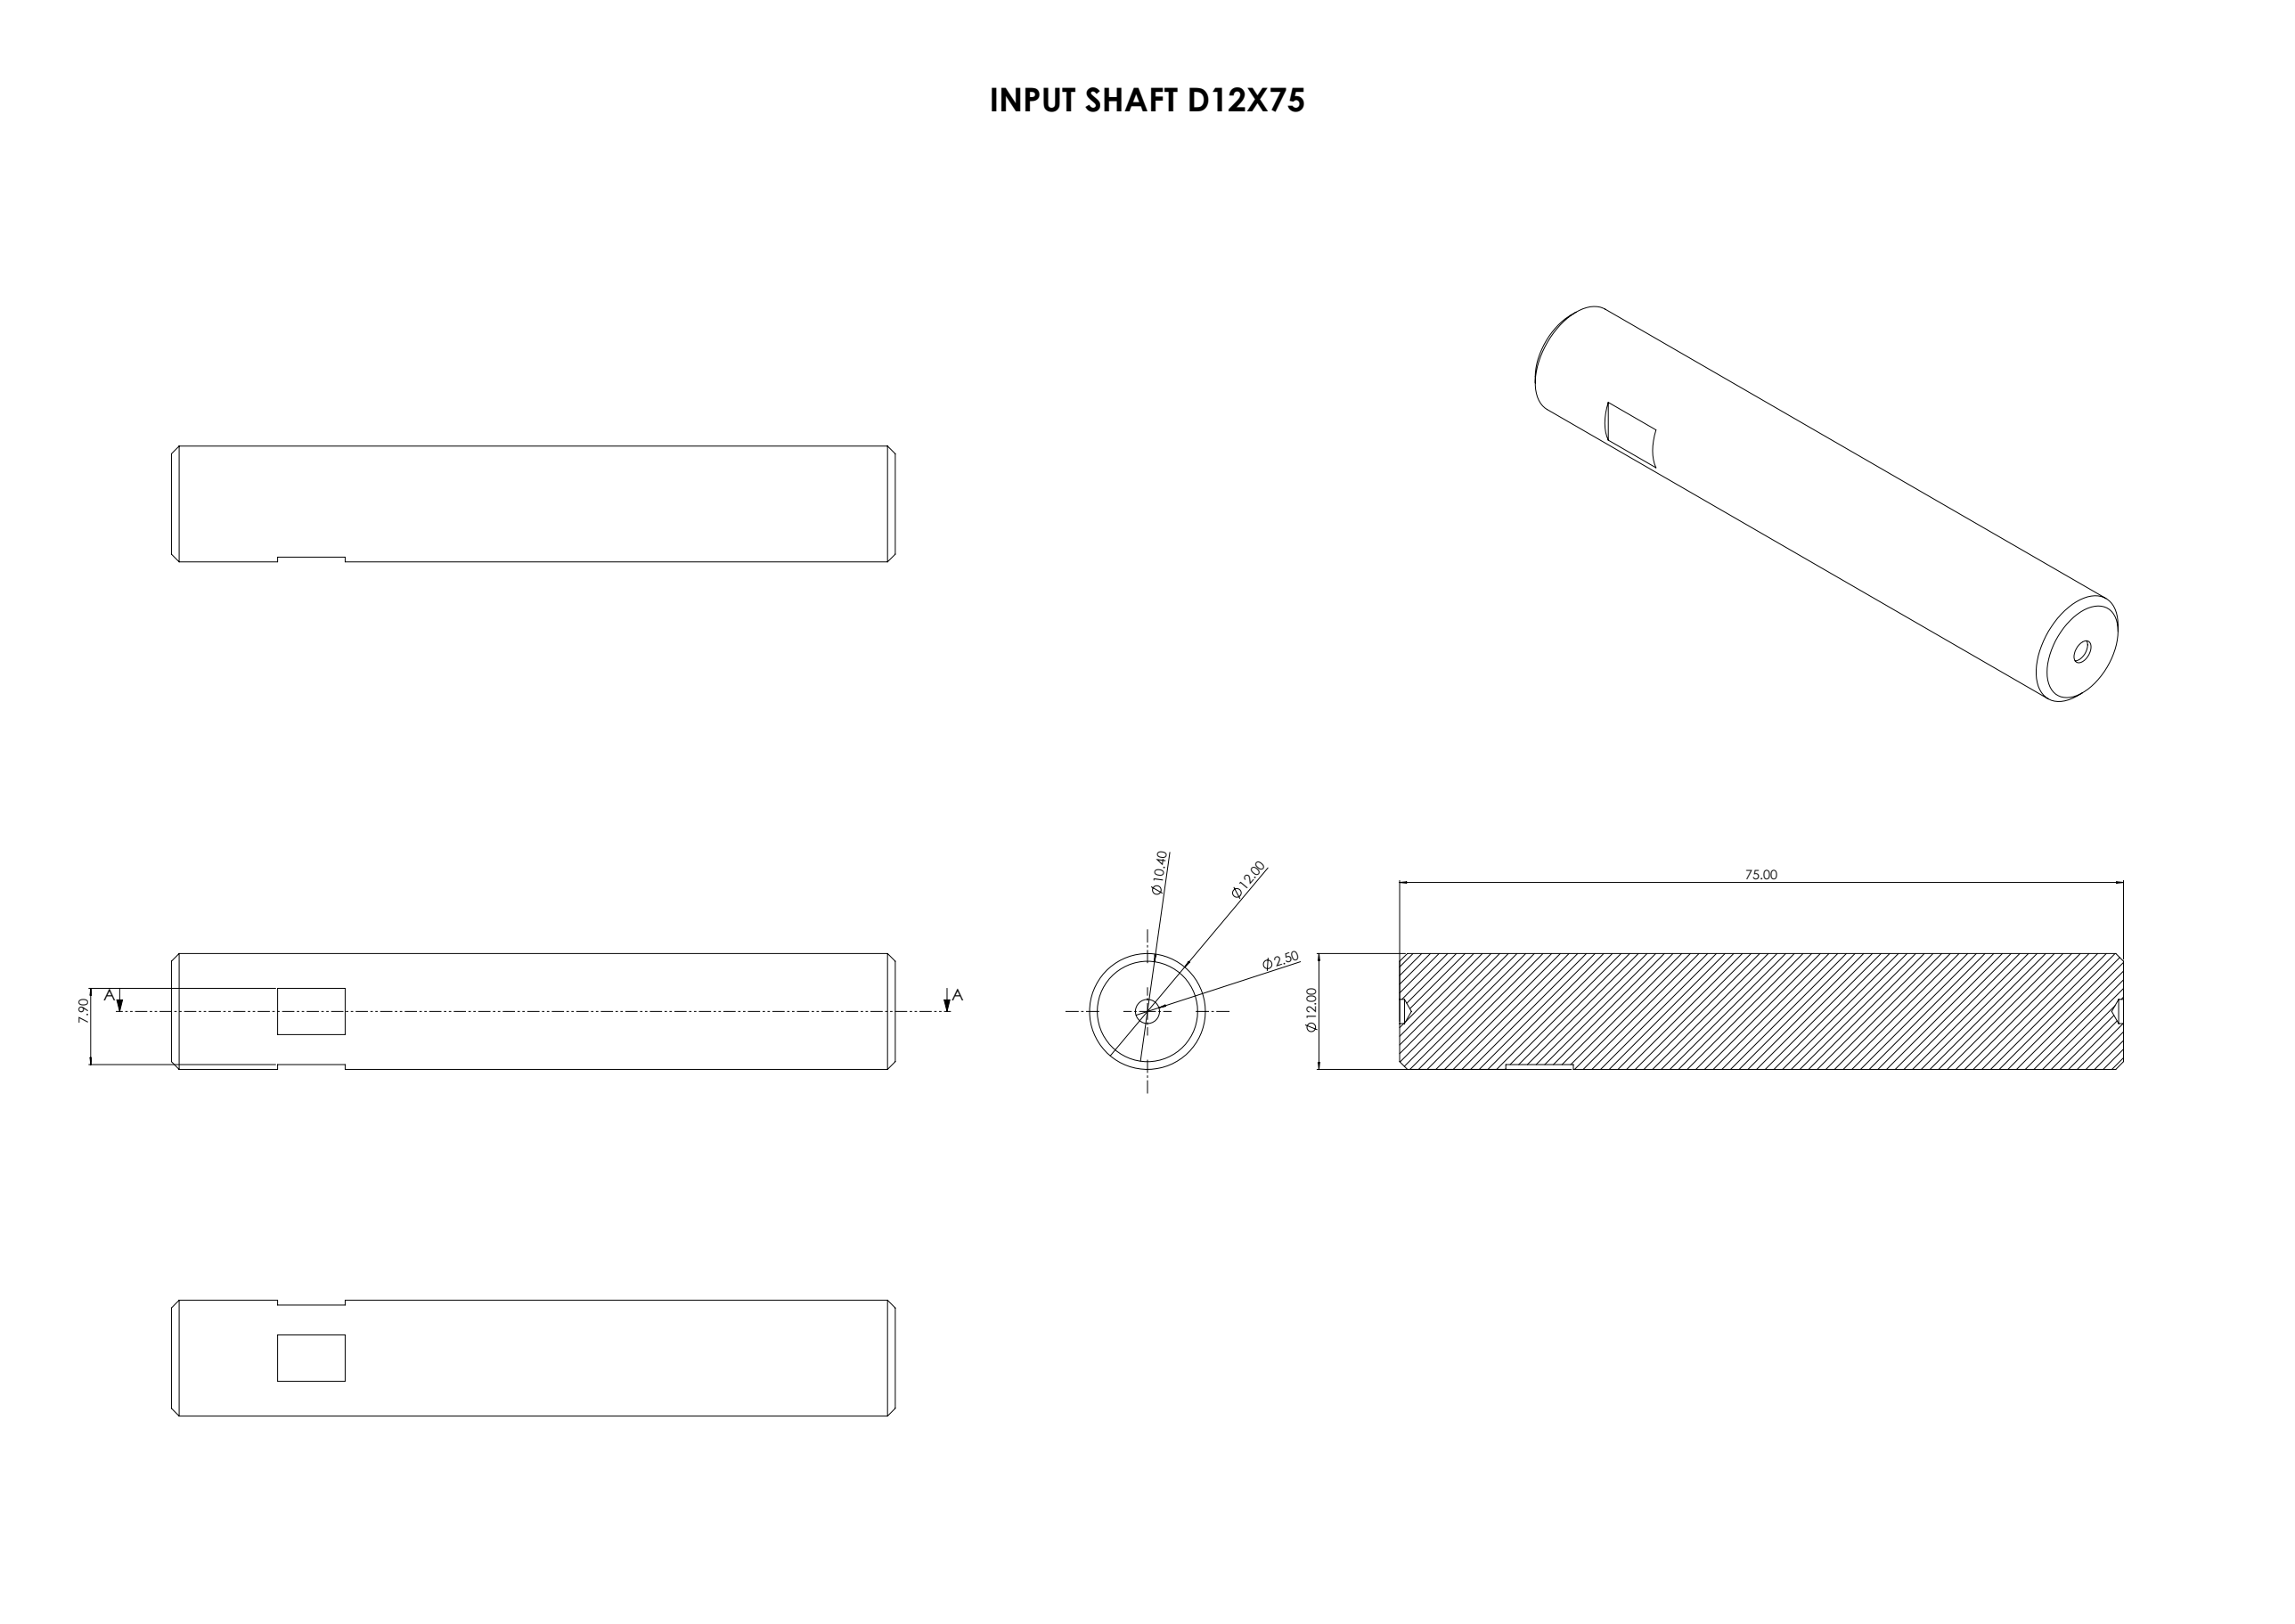
ISO-10303-21;
HEADER;
/* Generated by software containing ST-Developer
 * from STEP Tools, Inc. (www.steptools.com) 
 */

FILE_DESCRIPTION(
/* description */ (''),
/* implementation_level */ '2;1');

FILE_NAME(
/* name */ '04_Input_Shaft_D12x75.step',
/* time_stamp */ '2026-10-11T09:12:28-07:00',
/* author */ (''),
/* organization */ (''),
/* preprocessor_version */ 'ST-DEVELOPER v20.2',
/* originating_system */ 'Autodesk Translation Framework v15.15.0.0',
/* authorisation */ '');

FILE_SCHEMA (('AUTOMOTIVE_DESIGN { 1 0 10303 214 3 1 1 }'));
ENDSEC;

DATA;
#10=MECHANICAL_DESIGN_GEOMETRIC_PRESENTATION_REPRESENTATION('',(#650),#23254);
#630=SHAPE_REPRESENTATION_RELATIONSHIP('SRR','None',#23303,#640);
#640=ADVANCED_BREP_SHAPE_REPRESENTATION('',(#660),#23247);
#650=STYLED_ITEM('',(#23462),#660);
#660=MANIFOLD_SOLID_BREP('Body1',#7028);
#735=CONICAL_SURFACE('',#7557,0.625,1.04746029293308);
#736=CONICAL_SURFACE('',#7564,1.25,1.04746029293308);
#737=CONICAL_SURFACE('',#7567,5.6,0.785398163397448);
#738=CONICAL_SURFACE('',#7571,5.6,0.785398163397448);
#808=FACE_BOUND('',#1674,.T.);
#809=FACE_BOUND('',#1677,.T.);
#810=FACE_BOUND('',#1680,.T.);
#932=PLANE('',#7545);
#933=PLANE('',#7548);
#934=PLANE('',#7551);
#935=PLANE('',#7552);
#936=PLANE('',#7554);
#937=PLANE('',#7555);
#938=PLANE('',#7565);
#939=PLANE('',#7573);
#1240=FACE_OUTER_BOUND('',#1663,.T.);
#1241=FACE_OUTER_BOUND('',#1664,.T.);
#1242=FACE_OUTER_BOUND('',#1665,.T.);
#1243=FACE_OUTER_BOUND('',#1666,.T.);
#1244=FACE_OUTER_BOUND('',#1667,.T.);
#1245=FACE_OUTER_BOUND('',#1668,.T.);
#1246=FACE_OUTER_BOUND('',#1669,.T.);
#1247=FACE_OUTER_BOUND('',#1670,.T.);
#1248=FACE_OUTER_BOUND('',#1671,.T.);
#1249=FACE_OUTER_BOUND('',#1672,.T.);
#1250=FACE_OUTER_BOUND('',#1673,.T.);
#1251=FACE_OUTER_BOUND('',#1675,.T.);
#1252=FACE_OUTER_BOUND('',#1676,.T.);
#1253=FACE_OUTER_BOUND('',#1678,.T.);
#1254=FACE_OUTER_BOUND('',#1679,.T.);
#1663=EDGE_LOOP('',(#5873,#5874,#5875));
#1664=EDGE_LOOP('',(#5876,#5877,#5878));
#1665=EDGE_LOOP('',(#5879,#5880,#5881,#5882));
#1666=EDGE_LOOP('',(#5883,#5884));
#1667=EDGE_LOOP('',(#5885,#5886,#5887,#5888));
#1668=EDGE_LOOP('',(#5889,#5890));
#1669=EDGE_LOOP('',(#5891,#5892,#5893));
#1670=EDGE_LOOP('',(#5894,#5895,#5896,#5897));
#1671=EDGE_LOOP('',(#5898,#5899,#5900,#5901));
#1672=EDGE_LOOP('',(#5902,#5903,#5904));
#1673=EDGE_LOOP('',(#5905));
#1674=EDGE_LOOP('',(#5906));
#1675=EDGE_LOOP('',(#5907,#5908,#5909,#5910));
#1676=EDGE_LOOP('',(#5911,#5912,#5913,#5914,#5915,#5916,#5917,#5918,#5919,
#5920,#5921,#5922));
#1677=EDGE_LOOP('',(#5923,#5924,#5925,#5926));
#1678=EDGE_LOOP('',(#5927,#5928,#5929,#5930));
#1679=EDGE_LOOP('',(#5931));
#1680=EDGE_LOOP('',(#5932));
#1993=LINE('',#20982,#2252);
#1994=LINE('',#20989,#2253);
#1995=LINE('',#20992,#2254);
#1996=LINE('',#20993,#2255);
#1997=LINE('',#20998,#2256);
#1998=LINE('',#21001,#2257);
#1999=LINE('',#21003,#2258);
#2000=LINE('',#21004,#2259);
#2001=LINE('',#21010,#2260);
#2002=LINE('',#21014,#2261);
#2003=LINE('',#21020,#2262);
#2004=LINE('',#21024,#2263);
#2005=LINE('',#21031,#2264);
#2006=LINE('',#21035,#2265);
#2007=LINE('',#21036,#2266);
#2008=LINE('',#21040,#2267);
#2252=VECTOR('',#8785,10.);
#2253=VECTOR('',#8792,10.);
#2254=VECTOR('',#8797,10.);
#2255=VECTOR('',#8798,10.);
#2256=VECTOR('',#8803,10.);
#2257=VECTOR('',#8806,10.);
#2258=VECTOR('',#8807,10.);
#2259=VECTOR('',#8808,10.);
#2260=VECTOR('',#8815,0.625);
#2261=VECTOR('',#8820,1.25);
#2262=VECTOR('',#8827,1.25);
#2263=VECTOR('',#8832,1.25);
#2264=VECTOR('',#8841,5.6);
#2265=VECTOR('',#8846,6.);
#2266=VECTOR('',#8847,6.);
#2267=VECTOR('',#8852,5.6);
#2572=CIRCLE('',#7546,6.);
#2573=CIRCLE('',#7547,6.);
#2574=CIRCLE('',#7549,6.);
#2575=CIRCLE('',#7550,6.);
#2576=CIRCLE('',#7553,6.);
#2577=CIRCLE('',#7556,6.);
#2578=CIRCLE('',#7558,1.25);
#2579=CIRCLE('',#7560,1.25);
#2580=CIRCLE('',#7562,1.25);
#2581=CIRCLE('',#7563,1.25);
#2582=CIRCLE('',#7566,5.2);
#2583=CIRCLE('',#7568,6.);
#2584=CIRCLE('',#7570,6.);
#2585=CIRCLE('',#7572,5.2);
#3164=VERTEX_POINT('',#20978);
#3165=VERTEX_POINT('',#20979);
#3166=VERTEX_POINT('',#20981);
#3167=VERTEX_POINT('',#20985);
#3168=VERTEX_POINT('',#20986);
#3169=VERTEX_POINT('',#20988);
#3170=VERTEX_POINT('',#20995);
#3171=VERTEX_POINT('',#20996);
#3172=VERTEX_POINT('',#21000);
#3173=VERTEX_POINT('',#21002);
#3174=VERTEX_POINT('',#21008);
#3175=VERTEX_POINT('',#21009);
#3176=VERTEX_POINT('',#21013);
#3177=VERTEX_POINT('',#21017);
#3178=VERTEX_POINT('',#21019);
#3179=VERTEX_POINT('',#21023);
#3180=VERTEX_POINT('',#21026);
#3181=VERTEX_POINT('',#21029);
#3182=VERTEX_POINT('',#21033);
#3183=VERTEX_POINT('',#21038);
#4112=EDGE_CURVE('',#3164,#3165,#2572,.T.);
#4113=EDGE_CURVE('',#3164,#3166,#1993,.T.);
#4114=EDGE_CURVE('',#3165,#3166,#2573,.T.);
#4115=EDGE_CURVE('',#3167,#3168,#2574,.T.);
#4116=EDGE_CURVE('',#3167,#3169,#1994,.T.);
#4117=EDGE_CURVE('',#3168,#3169,#2575,.T.);
#4118=EDGE_CURVE('',#3169,#3164,#1995,.T.);
#4119=EDGE_CURVE('',#3166,#3167,#1996,.T.);
#4120=EDGE_CURVE('',#3170,#3171,#2576,.T.);
#4121=EDGE_CURVE('',#3170,#3171,#1997,.T.);
#4122=EDGE_CURVE('',#3172,#3170,#1998,.T.);
#4123=EDGE_CURVE('',#3173,#3172,#1999,.T.);
#4124=EDGE_CURVE('',#3171,#3173,#2000,.T.);
#4125=EDGE_CURVE('',#3173,#3172,#2577,.T.);
#4126=EDGE_CURVE('',#3174,#3175,#2001,.T.);
#4127=EDGE_CURVE('',#3175,#3175,#2578,.T.);
#4128=EDGE_CURVE('',#3175,#3176,#2002,.T.);
#4129=EDGE_CURVE('',#3176,#3176,#2579,.T.);
#4130=EDGE_CURVE('',#3177,#3177,#2580,.T.);
#4131=EDGE_CURVE('',#3177,#3178,#2003,.T.);
#4132=EDGE_CURVE('',#3178,#3178,#2581,.T.);
#4133=EDGE_CURVE('',#3178,#3179,#2004,.T.);
#4134=EDGE_CURVE('',#3180,#3180,#2582,.T.);
#4135=EDGE_CURVE('',#3181,#3181,#2583,.T.);
#4136=EDGE_CURVE('',#3181,#3180,#2005,.T.);
#4137=EDGE_CURVE('',#3182,#3182,#2584,.T.);
#4138=EDGE_CURVE('',#3182,#3168,#2006,.T.);
#4139=EDGE_CURVE('',#3165,#3181,#2007,.T.);
#4140=EDGE_CURVE('',#3183,#3183,#2585,.T.);
#4141=EDGE_CURVE('',#3183,#3182,#2008,.T.);
#5873=ORIENTED_EDGE('',*,*,#4112,.F.);
#5874=ORIENTED_EDGE('',*,*,#4113,.T.);
#5875=ORIENTED_EDGE('',*,*,#4114,.F.);
#5876=ORIENTED_EDGE('',*,*,#4115,.F.);
#5877=ORIENTED_EDGE('',*,*,#4116,.T.);
#5878=ORIENTED_EDGE('',*,*,#4117,.F.);
#5879=ORIENTED_EDGE('',*,*,#4118,.F.);
#5880=ORIENTED_EDGE('',*,*,#4116,.F.);
#5881=ORIENTED_EDGE('',*,*,#4119,.F.);
#5882=ORIENTED_EDGE('',*,*,#4113,.F.);
#5883=ORIENTED_EDGE('',*,*,#4120,.F.);
#5884=ORIENTED_EDGE('',*,*,#4121,.T.);
#5885=ORIENTED_EDGE('',*,*,#4122,.F.);
#5886=ORIENTED_EDGE('',*,*,#4123,.F.);
#5887=ORIENTED_EDGE('',*,*,#4124,.F.);
#5888=ORIENTED_EDGE('',*,*,#4121,.F.);
#5889=ORIENTED_EDGE('',*,*,#4125,.F.);
#5890=ORIENTED_EDGE('',*,*,#4123,.T.);
#5891=ORIENTED_EDGE('',*,*,#4126,.T.);
#5892=ORIENTED_EDGE('',*,*,#4127,.T.);
#5893=ORIENTED_EDGE('',*,*,#4126,.F.);
#5894=ORIENTED_EDGE('',*,*,#4127,.F.);
#5895=ORIENTED_EDGE('',*,*,#4128,.T.);
#5896=ORIENTED_EDGE('',*,*,#4129,.F.);
#5897=ORIENTED_EDGE('',*,*,#4128,.F.);
#5898=ORIENTED_EDGE('',*,*,#4130,.F.);
#5899=ORIENTED_EDGE('',*,*,#4131,.T.);
#5900=ORIENTED_EDGE('',*,*,#4132,.T.);
#5901=ORIENTED_EDGE('',*,*,#4131,.F.);
#5902=ORIENTED_EDGE('',*,*,#4132,.F.);
#5903=ORIENTED_EDGE('',*,*,#4133,.T.);
#5904=ORIENTED_EDGE('',*,*,#4133,.F.);
#5905=ORIENTED_EDGE('',*,*,#4134,.F.);
#5906=ORIENTED_EDGE('',*,*,#4130,.T.);
#5907=ORIENTED_EDGE('',*,*,#4135,.F.);
#5908=ORIENTED_EDGE('',*,*,#4136,.T.);
#5909=ORIENTED_EDGE('',*,*,#4134,.T.);
#5910=ORIENTED_EDGE('',*,*,#4136,.F.);
#5911=ORIENTED_EDGE('',*,*,#4137,.F.);
#5912=ORIENTED_EDGE('',*,*,#4138,.T.);
#5913=ORIENTED_EDGE('',*,*,#4117,.T.);
#5914=ORIENTED_EDGE('',*,*,#4118,.T.);
#5915=ORIENTED_EDGE('',*,*,#4112,.T.);
#5916=ORIENTED_EDGE('',*,*,#4139,.T.);
#5917=ORIENTED_EDGE('',*,*,#4135,.T.);
#5918=ORIENTED_EDGE('',*,*,#4139,.F.);
#5919=ORIENTED_EDGE('',*,*,#4114,.T.);
#5920=ORIENTED_EDGE('',*,*,#4119,.T.);
#5921=ORIENTED_EDGE('',*,*,#4115,.T.);
#5922=ORIENTED_EDGE('',*,*,#4138,.F.);
#5923=ORIENTED_EDGE('',*,*,#4124,.T.);
#5924=ORIENTED_EDGE('',*,*,#4125,.T.);
#5925=ORIENTED_EDGE('',*,*,#4122,.T.);
#5926=ORIENTED_EDGE('',*,*,#4120,.T.);
#5927=ORIENTED_EDGE('',*,*,#4140,.F.);
#5928=ORIENTED_EDGE('',*,*,#4141,.T.);
#5929=ORIENTED_EDGE('',*,*,#4137,.T.);
#5930=ORIENTED_EDGE('',*,*,#4141,.F.);
#5931=ORIENTED_EDGE('',*,*,#4140,.T.);
#5932=ORIENTED_EDGE('',*,*,#4129,.T.);
#6599=CYLINDRICAL_SURFACE('',#7559,1.25);
#6600=CYLINDRICAL_SURFACE('',#7561,1.25);
#6601=CYLINDRICAL_SURFACE('',#7569,6.);
#6891=ADVANCED_FACE('',(#1240),#932,.F.);
#6892=ADVANCED_FACE('',(#1241),#933,.F.);
#6893=ADVANCED_FACE('',(#1242),#934,.F.);
#6894=ADVANCED_FACE('',(#1243),#935,.F.);
#6895=ADVANCED_FACE('',(#1244),#936,.F.);
#6896=ADVANCED_FACE('',(#1245),#937,.F.);
#6897=ADVANCED_FACE('',(#1246),#735,.F.);
#6898=ADVANCED_FACE('',(#1247),#6599,.F.);
#6899=ADVANCED_FACE('',(#1248),#6600,.F.);
#6900=ADVANCED_FACE('',(#1249),#736,.F.);
#6901=ADVANCED_FACE('',(#1250,#808),#938,.T.);
#6902=ADVANCED_FACE('',(#1251),#737,.T.);
#6903=ADVANCED_FACE('',(#1252,#809),#6601,.T.);
#6904=ADVANCED_FACE('',(#1253),#738,.T.);
#6905=ADVANCED_FACE('',(#1254,#810),#939,.T.);
#7028=CLOSED_SHELL('',(#6891,#6892,#6893,#6894,#6895,#6896,#6897,#6898,
#6899,#6900,#6901,#6902,#6903,#6904,#6905));
#7544=AXIS2_PLACEMENT_3D('',#20976,#8779,#8780);
#7545=AXIS2_PLACEMENT_3D('',#20977,#8781,#8782);
#7546=AXIS2_PLACEMENT_3D('',#20980,#8783,#8784);
#7547=AXIS2_PLACEMENT_3D('',#20983,#8786,#8787);
#7548=AXIS2_PLACEMENT_3D('',#20984,#8788,#8789);
#7549=AXIS2_PLACEMENT_3D('',#20987,#8790,#8791);
#7550=AXIS2_PLACEMENT_3D('',#20990,#8793,#8794);
#7551=AXIS2_PLACEMENT_3D('',#20991,#8795,#8796);
#7552=AXIS2_PLACEMENT_3D('',#20994,#8799,#8800);
#7553=AXIS2_PLACEMENT_3D('',#20997,#8801,#8802);
#7554=AXIS2_PLACEMENT_3D('',#20999,#8804,#8805);
#7555=AXIS2_PLACEMENT_3D('',#21005,#8809,#8810);
#7556=AXIS2_PLACEMENT_3D('',#21006,#8811,#8812);
#7557=AXIS2_PLACEMENT_3D('',#21007,#8813,#8814);
#7558=AXIS2_PLACEMENT_3D('',#21011,#8816,#8817);
#7559=AXIS2_PLACEMENT_3D('',#21012,#8818,#8819);
#7560=AXIS2_PLACEMENT_3D('',#21015,#8821,#8822);
#7561=AXIS2_PLACEMENT_3D('',#21016,#8823,#8824);
#7562=AXIS2_PLACEMENT_3D('',#21018,#8825,#8826);
#7563=AXIS2_PLACEMENT_3D('',#21021,#8828,#8829);
#7564=AXIS2_PLACEMENT_3D('',#21022,#8830,#8831);
#7565=AXIS2_PLACEMENT_3D('',#21025,#8833,#8834);
#7566=AXIS2_PLACEMENT_3D('',#21027,#8835,#8836);
#7567=AXIS2_PLACEMENT_3D('',#21028,#8837,#8838);
#7568=AXIS2_PLACEMENT_3D('',#21030,#8839,#8840);
#7569=AXIS2_PLACEMENT_3D('',#21032,#8842,#8843);
#7570=AXIS2_PLACEMENT_3D('',#21034,#8844,#8845);
#7571=AXIS2_PLACEMENT_3D('',#21037,#8848,#8849);
#7572=AXIS2_PLACEMENT_3D('',#21039,#8850,#8851);
#7573=AXIS2_PLACEMENT_3D('',#21041,#8853,#8854);
#8779=DIRECTION('axis',(0.,0.,1.));
#8780=DIRECTION('refdir',(1.,0.,0.));
#8781=DIRECTION('center_axis',(-1.,0.,0.));
#8782=DIRECTION('ref_axis',(0.,0.,1.));
#8783=DIRECTION('center_axis',(-1.,0.,0.));
#8784=DIRECTION('ref_axis',(0.,1.,0.));
#8785=DIRECTION('',(0.,0.,1.));
#8786=DIRECTION('center_axis',(-1.,0.,0.));
#8787=DIRECTION('ref_axis',(0.,1.,0.));
#8788=DIRECTION('center_axis',(1.,0.,0.));
#8789=DIRECTION('ref_axis',(0.,0.,-1.));
#8790=DIRECTION('center_axis',(1.,0.,0.));
#8791=DIRECTION('ref_axis',(0.,1.,0.));
#8792=DIRECTION('',(0.,0.,-1.));
#8793=DIRECTION('center_axis',(1.,0.,0.));
#8794=DIRECTION('ref_axis',(0.,1.,0.));
#8795=DIRECTION('center_axis',(0.,1.,0.));
#8796=DIRECTION('ref_axis',(0.,0.,1.));
#8797=DIRECTION('',(-1.,0.,0.));
#8798=DIRECTION('',(1.,0.,0.));
#8799=DIRECTION('center_axis',(-1.,0.,0.));
#8800=DIRECTION('ref_axis',(0.,-1.,0.));
#8801=DIRECTION('center_axis',(-1.,0.,0.));
#8802=DIRECTION('ref_axis',(0.,1.,0.));
#8803=DIRECTION('',(0.,1.,0.));
#8804=DIRECTION('center_axis',(0.,0.,-1.));
#8805=DIRECTION('ref_axis',(-1.,0.,0.));
#8806=DIRECTION('',(-1.,0.,0.));
#8807=DIRECTION('',(0.,-1.,0.));
#8808=DIRECTION('',(1.,0.,0.));
#8809=DIRECTION('center_axis',(1.,0.,0.));
#8810=DIRECTION('ref_axis',(0.,1.,0.));
#8811=DIRECTION('center_axis',(1.,0.,0.));
#8812=DIRECTION('ref_axis',(0.,1.,0.));
#8813=DIRECTION('center_axis',(1.,0.,0.));
#8814=DIRECTION('ref_axis',(0.,1.,0.));
#8815=DIRECTION('',(0.499772441725887,-0.866156744758906,-1.06073608502889E-16));
#8816=DIRECTION('center_axis',(1.,0.,0.));
#8817=DIRECTION('ref_axis',(0.,0.,-1.));
#8818=DIRECTION('center_axis',(1.,0.,0.));
#8819=DIRECTION('ref_axis',(0.,1.,0.));
#8820=DIRECTION('',(1.,0.,0.));
#8821=DIRECTION('center_axis',(-1.,0.,0.));
#8822=DIRECTION('ref_axis',(0.,1.,0.));
#8823=DIRECTION('center_axis',(1.,0.,0.));
#8824=DIRECTION('ref_axis',(0.,1.,0.));
#8825=DIRECTION('center_axis',(1.,0.,0.));
#8826=DIRECTION('ref_axis',(0.,1.,0.));
#8827=DIRECTION('',(1.,0.,0.));
#8828=DIRECTION('center_axis',(1.,0.,0.));
#8829=DIRECTION('ref_axis',(0.,0.,-1.));
#8830=DIRECTION('center_axis',(-1.,0.,0.));
#8831=DIRECTION('ref_axis',(0.,1.,0.));
#8832=DIRECTION('',(0.499772441725888,0.866156744758905,1.06073608502888E-16));
#8833=DIRECTION('center_axis',(-1.,0.,0.));
#8834=DIRECTION('ref_axis',(0.,0.,1.));
#8835=DIRECTION('center_axis',(1.,0.,0.));
#8836=DIRECTION('ref_axis',(0.,0.,-1.));
#8837=DIRECTION('center_axis',(1.,0.,0.));
#8838=DIRECTION('ref_axis',(0.,1.,0.));
#8839=DIRECTION('center_axis',(1.,0.,0.));
#8840=DIRECTION('ref_axis',(0.,0.,-1.));
#8841=DIRECTION('',(-0.707106781186548,0.707106781186547,8.65956056235493E-17));
#8842=DIRECTION('center_axis',(1.,0.,0.));
#8843=DIRECTION('ref_axis',(0.,1.,0.));
#8844=DIRECTION('center_axis',(1.,0.,0.));
#8845=DIRECTION('ref_axis',(0.,0.,-1.));
#8846=DIRECTION('',(-1.,0.,0.));
#8847=DIRECTION('',(-1.,0.,0.));
#8848=DIRECTION('center_axis',(-1.,0.,0.));
#8849=DIRECTION('ref_axis',(0.,1.,0.));
#8850=DIRECTION('center_axis',(1.,0.,0.));
#8851=DIRECTION('ref_axis',(0.,0.,-1.));
#8852=DIRECTION('',(-0.707106781186548,-0.707106781186547,-8.65956056235493E-17));
#8853=DIRECTION('center_axis',(1.,0.,0.));
#8854=DIRECTION('ref_axis',(0.,0.,-1.));
#20976=CARTESIAN_POINT('',(0.,0.,0.));
#20977=CARTESIAN_POINT('Origin',(21.,-6.,-7.));
#20978=CARTESIAN_POINT('',(21.,-5.5,-2.39791576165636));
#20979=CARTESIAN_POINT('',(21.,-6.,-7.34788079488412E-16));
#20980=CARTESIAN_POINT('Origin',(21.,0.,0.));
#20981=CARTESIAN_POINT('',(21.,-5.5,2.39791576165636));
#20982=CARTESIAN_POINT('',(21.,-5.5,7.));
#20983=CARTESIAN_POINT('Origin',(21.,0.,0.));
#20984=CARTESIAN_POINT('Origin',(28.,-6.,7.));
#20985=CARTESIAN_POINT('',(28.,-5.5,2.39791576165636));
#20986=CARTESIAN_POINT('',(28.,-6.,-7.34788079488412E-16));
#20987=CARTESIAN_POINT('Origin',(28.,0.,0.));
#20988=CARTESIAN_POINT('',(28.,-5.5,-2.39791576165636));
#20989=CARTESIAN_POINT('',(28.,-5.5,-7.));
#20990=CARTESIAN_POINT('Origin',(28.,0.,0.));
#20991=CARTESIAN_POINT('Origin',(24.5,-5.5,0.));
#20992=CARTESIAN_POINT('',(47.5,-5.5,-2.39791576165636));
#20993=CARTESIAN_POINT('',(47.5,-5.5,2.39791576165636));
#20994=CARTESIAN_POINT('Origin',(21.,7.,6.));
#20995=CARTESIAN_POINT('',(21.,-2.39791576165636,5.5));
#20996=CARTESIAN_POINT('',(21.,2.39791576165636,5.5));
#20997=CARTESIAN_POINT('Origin',(21.,0.,0.));
#20998=CARTESIAN_POINT('',(21.,7.,5.5));
#20999=CARTESIAN_POINT('Origin',(24.5,0.,5.5));
#21000=CARTESIAN_POINT('',(28.,-2.39791576165636,5.5));
#21001=CARTESIAN_POINT('',(47.5,-2.39791576165636,5.5));
#21002=CARTESIAN_POINT('',(28.,2.39791576165636,5.5));
#21003=CARTESIAN_POINT('',(28.,-7.,5.5));
#21004=CARTESIAN_POINT('',(47.5,2.39791576165636,5.5));
#21005=CARTESIAN_POINT('Origin',(28.,-7.,6.));
#21006=CARTESIAN_POINT('Origin',(28.,0.,0.));
#21007=CARTESIAN_POINT('Origin',(84.139375,0.,0.));
#21008=CARTESIAN_POINT('',(83.77875,0.,0.));
#21009=CARTESIAN_POINT('',(84.5,-1.25,-1.53080849893419E-16));
#21010=CARTESIAN_POINT('',(84.139375,-0.625,-7.65404249467096E-17));
#21011=CARTESIAN_POINT('Origin',(84.5,0.,0.));
#21012=CARTESIAN_POINT('Origin',(84.75,0.,0.));
#21013=CARTESIAN_POINT('',(85.,-1.25,-1.53080849893419E-16));
#21014=CARTESIAN_POINT('',(84.75,-1.25,-1.53080849893419E-16));
#21015=CARTESIAN_POINT('Origin',(85.,0.,0.));
#21016=CARTESIAN_POINT('Origin',(10.25,0.,0.));
#21017=CARTESIAN_POINT('',(10.,-1.25,-1.53080849893419E-16));
#21018=CARTESIAN_POINT('Origin',(10.,0.,0.));
#21019=CARTESIAN_POINT('',(10.5,-1.25,-1.53080849893419E-16));
#21020=CARTESIAN_POINT('',(10.25,-1.25,-1.53080849893419E-16));
#21021=CARTESIAN_POINT('Origin',(10.5,0.,0.));
#21022=CARTESIAN_POINT('Origin',(10.5,0.,0.));
#21023=CARTESIAN_POINT('',(11.22125,0.,0.));
#21024=CARTESIAN_POINT('',(10.5,-1.25,-1.53080849893419E-16));
#21025=CARTESIAN_POINT('Origin',(10.,5.2,0.));
#21026=CARTESIAN_POINT('',(10.,-5.2,-6.36816335556624E-16));
#21027=CARTESIAN_POINT('Origin',(10.,0.,0.));
#21028=CARTESIAN_POINT('Origin',(10.4,0.,0.));
#21029=CARTESIAN_POINT('',(10.8,-6.,-7.34788079488412E-16));
#21030=CARTESIAN_POINT('Origin',(10.8,0.,0.));
#21031=CARTESIAN_POINT('',(10.4,-5.6,-6.85802207522518E-16));
#21032=CARTESIAN_POINT('Origin',(47.5,0.,0.));
#21033=CARTESIAN_POINT('',(84.2,-6.,-7.34788079488412E-16));
#21034=CARTESIAN_POINT('Origin',(84.2,0.,0.));
#21035=CARTESIAN_POINT('',(47.5,-6.,-7.34788079488412E-16));
#21036=CARTESIAN_POINT('',(47.5,-6.,-7.34788079488412E-16));
#21037=CARTESIAN_POINT('Origin',(84.6,0.,0.));
#21038=CARTESIAN_POINT('',(85.,-5.2,-6.36816335556624E-16));
#21039=CARTESIAN_POINT('Origin',(85.,0.,0.));
#21040=CARTESIAN_POINT('',(84.6,-5.6,-6.85802207522518E-16));
#21041=CARTESIAN_POINT('Origin',(85.,0.,0.));
#23235=UNCERTAINTY_MEASURE_WITH_UNIT(LENGTH_MEASURE(0.01),#23255,
'DISTANCE_ACCURACY_VALUE',
'Maximum model space distance between geometric entities at asserted c
onnectivities');
#23242=UNCERTAINTY_MEASURE_WITH_UNIT(LENGTH_MEASURE(0.01),#23255,
'DISTANCE_ACCURACY_VALUE',
'Maximum model space distance between geometric entities at asserted c
onnectivities');
#23247=(
GEOMETRIC_REPRESENTATION_CONTEXT(3)
GLOBAL_UNCERTAINTY_ASSIGNED_CONTEXT((#23235))
GLOBAL_UNIT_ASSIGNED_CONTEXT((#23255,#23257,#23258))
REPRESENTATION_CONTEXT('','3D')
);
#23254=(
GEOMETRIC_REPRESENTATION_CONTEXT(3)
GLOBAL_UNCERTAINTY_ASSIGNED_CONTEXT((#23242))
GLOBAL_UNIT_ASSIGNED_CONTEXT((#23255,#23257,#23258))
REPRESENTATION_CONTEXT('','3D')
);
#23255=(
LENGTH_UNIT()
NAMED_UNIT(*)
SI_UNIT(.MILLI.,.METRE.)
);
#23257=(
NAMED_UNIT(*)
PLANE_ANGLE_UNIT()
SI_UNIT($,.RADIAN.)
);
#23258=(
NAMED_UNIT(*)
SI_UNIT($,.STERADIAN.)
SOLID_ANGLE_UNIT()
);
#23263=SHAPE_DEFINITION_REPRESENTATION(#23274,#23303);
#23274=PRODUCT_DEFINITION_SHAPE('',$,#23315);
#23303=SHAPE_REPRESENTATION('',(#7544),#23247);
#23310=PRODUCT_DEFINITION_CONTEXT('part definition',#23345,'design');
#23315=PRODUCT_DEFINITION('2026-10-11-09-11-51-553',
'04_Input_Shaft_D12x75',#23326,#23310);
#23326=PRODUCT_DEFINITION_FORMATION('',$,#23351);
#23345=APPLICATION_CONTEXT(
'Core Data for Automotive Mechanical Design Process');
#23346=PRODUCT_CONTEXT('part definition',#23345,'mechanical');
#23351=PRODUCT('2026-10-11-09-11-51-553','04_Input_Shaft_D12x75',$,(#23346));
#23456=COLOUR_RGB('Grey',0.48,0.52,0.57);
#23457=FILL_AREA_STYLE_COLOUR('',#23456);
#23458=FILL_AREA_STYLE('',(#23457));
#23459=SURFACE_STYLE_FILL_AREA(#23458);
#23460=SURFACE_SIDE_STYLE('',(#23459));
#23461=SURFACE_STYLE_USAGE(.BOTH.,#23460);
#23462=PRESENTATION_STYLE_ASSIGNMENT((#23461));
ENDSEC;
END-ISO-10303-21;
